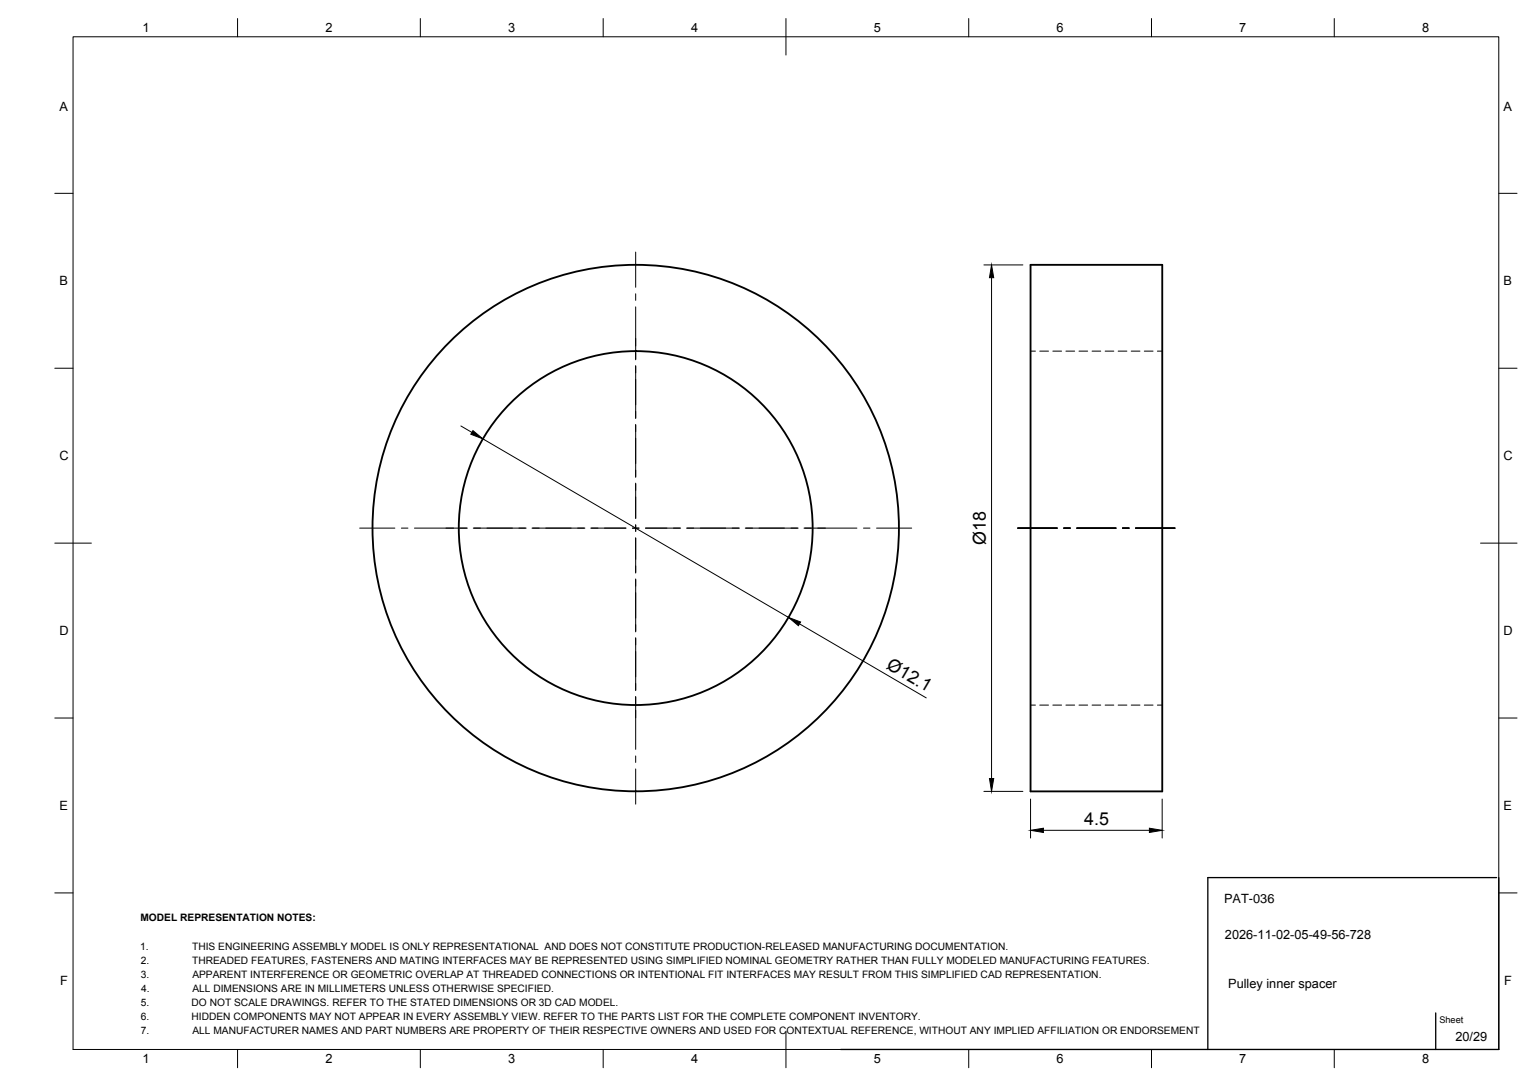
ISO-10303-21;
HEADER;
/* Generated by software containing ST-Developer
 * from STEP Tools, Inc. (www.steptools.com) 
 */

FILE_DESCRIPTION(
/* description */ ('Flange-mounted spindle'),
/* implementation_level */ '2;1');

FILE_NAME(
/* name */ 'Pulley inner spacer.step',
/* time_stamp */ '2026-10-27T10:49:51-07:00',
/* author */ (''),
/* organization */ (''),
/* preprocessor_version */ 'ST-DEVELOPER v20.2',
/* originating_system */ 'Autodesk Translation Framework v15.17.0.0',
/* authorisation */ '');

FILE_SCHEMA (('AUTOMOTIVE_DESIGN { 1 0 10303 214 3 1 1 }'));
ENDSEC;

DATA;
#10=MECHANICAL_DESIGN_GEOMETRIC_PRESENTATION_REPRESENTATION('',(#352),#11764);
#297=SHAPE_REPRESENTATION_RELATIONSHIP('SRR','None',#11895,#324);
#324=ADVANCED_BREP_SHAPE_REPRESENTATION('',(#378),#11750);
#352=STYLED_ITEM('',(#12113),#378);
#378=MANIFOLD_SOLID_BREP('Body1',#6146);
#457=FACE_BOUND('',#1228,.T.);
#458=FACE_BOUND('',#1230,.T.);
#594=PLANE('',#6714);
#595=PLANE('',#6715);
#814=FACE_OUTER_BOUND('',#1225,.T.);
#815=FACE_OUTER_BOUND('',#1226,.T.);
#816=FACE_OUTER_BOUND('',#1227,.T.);
#817=FACE_OUTER_BOUND('',#1229,.T.);
#1225=EDGE_LOOP('',(#4599,#4600,#4601,#4602));
#1226=EDGE_LOOP('',(#4603,#4604,#4605,#4606));
#1227=EDGE_LOOP('',(#4607));
#1228=EDGE_LOOP('',(#4608));
#1229=EDGE_LOOP('',(#4609));
#1230=EDGE_LOOP('',(#4610));
#1663=LINE('',#10200,#2085);
#1664=LINE('',#10206,#2086);
#2085=VECTOR('',#7894,0.605);
#2086=VECTOR('',#7901,0.9);
#2412=CIRCLE('',#6709,0.605);
#2413=CIRCLE('',#6710,0.605);
#2414=CIRCLE('',#6712,0.9);
#2415=CIRCLE('',#6713,0.9);
#2852=VERTEX_POINT('',#10197);
#2853=VERTEX_POINT('',#10199);
#2854=VERTEX_POINT('',#10203);
#2855=VERTEX_POINT('',#10205);
#3492=EDGE_CURVE('',#2852,#2852,#2412,.T.);
#3493=EDGE_CURVE('',#2852,#2853,#1663,.T.);
#3494=EDGE_CURVE('',#2853,#2853,#2413,.T.);
#3495=EDGE_CURVE('',#2854,#2854,#2414,.T.);
#3496=EDGE_CURVE('',#2854,#2855,#1664,.T.);
#3497=EDGE_CURVE('',#2855,#2855,#2415,.T.);
#4599=ORIENTED_EDGE('',*,*,#3492,.F.);
#4600=ORIENTED_EDGE('',*,*,#3493,.T.);
#4601=ORIENTED_EDGE('',*,*,#3494,.T.);
#4602=ORIENTED_EDGE('',*,*,#3493,.F.);
#4603=ORIENTED_EDGE('',*,*,#3495,.F.);
#4604=ORIENTED_EDGE('',*,*,#3496,.T.);
#4605=ORIENTED_EDGE('',*,*,#3497,.T.);
#4606=ORIENTED_EDGE('',*,*,#3496,.F.);
#4607=ORIENTED_EDGE('',*,*,#3495,.T.);
#4608=ORIENTED_EDGE('',*,*,#3492,.T.);
#4609=ORIENTED_EDGE('',*,*,#3497,.F.);
#4610=ORIENTED_EDGE('',*,*,#3494,.F.);
#5668=CYLINDRICAL_SURFACE('',#6708,0.605);
#5669=CYLINDRICAL_SURFACE('',#6711,0.9);
#5925=ADVANCED_FACE('',(#814),#5668,.F.);
#5926=ADVANCED_FACE('',(#815),#5669,.T.);
#5927=ADVANCED_FACE('',(#816,#457),#594,.T.);
#5928=ADVANCED_FACE('',(#817,#458),#595,.F.);
#6146=CLOSED_SHELL('',(#5925,#5926,#5927,#5928));
#6707=AXIS2_PLACEMENT_3D('',#10195,#7888,#7889);
#6708=AXIS2_PLACEMENT_3D('',#10196,#7890,#7891);
#6709=AXIS2_PLACEMENT_3D('',#10198,#7892,#7893);
#6710=AXIS2_PLACEMENT_3D('',#10201,#7895,#7896);
#6711=AXIS2_PLACEMENT_3D('',#10202,#7897,#7898);
#6712=AXIS2_PLACEMENT_3D('',#10204,#7899,#7900);
#6713=AXIS2_PLACEMENT_3D('',#10207,#7902,#7903);
#6714=AXIS2_PLACEMENT_3D('',#10208,#7904,#7905);
#6715=AXIS2_PLACEMENT_3D('',#10209,#7906,#7907);
#7888=DIRECTION('axis',(0.,0.,1.));
#7889=DIRECTION('refdir',(1.,0.,0.));
#7890=DIRECTION('center_axis',(0.,1.,0.));
#7891=DIRECTION('ref_axis',(1.,0.,0.));
#7892=DIRECTION('center_axis',(0.,-1.,0.));
#7893=DIRECTION('ref_axis',(1.,0.,0.));
#7894=DIRECTION('',(0.,-1.,0.));
#7895=DIRECTION('center_axis',(0.,-1.,0.));
#7896=DIRECTION('ref_axis',(1.,0.,0.));
#7897=DIRECTION('center_axis',(0.,1.,0.));
#7898=DIRECTION('ref_axis',(1.,0.,0.));
#7899=DIRECTION('center_axis',(0.,1.,0.));
#7900=DIRECTION('ref_axis',(1.,0.,0.));
#7901=DIRECTION('',(0.,-1.,0.));
#7902=DIRECTION('center_axis',(0.,1.,0.));
#7903=DIRECTION('ref_axis',(1.,0.,0.));
#7904=DIRECTION('center_axis',(0.,1.,0.));
#7905=DIRECTION('ref_axis',(1.,0.,0.));
#7906=DIRECTION('center_axis',(0.,1.,0.));
#7907=DIRECTION('ref_axis',(1.,0.,0.));
#10195=CARTESIAN_POINT('',(0.,0.,0.));
#10196=CARTESIAN_POINT('Origin',(0.,-4.95,8.));
#10197=CARTESIAN_POINT('',(-0.605,-4.5,8.));
#10198=CARTESIAN_POINT('Origin',(0.,-4.5,8.));
#10199=CARTESIAN_POINT('',(-0.605,-4.95,8.));
#10200=CARTESIAN_POINT('',(-0.605,-4.95,8.));
#10201=CARTESIAN_POINT('Origin',(0.,-4.95,8.));
#10202=CARTESIAN_POINT('Origin',(0.,-4.95,8.));
#10203=CARTESIAN_POINT('',(-0.9,-4.5,8.));
#10204=CARTESIAN_POINT('Origin',(0.,-4.5,8.));
#10205=CARTESIAN_POINT('',(-0.9,-4.95,8.));
#10206=CARTESIAN_POINT('',(-0.9,-4.95,8.));
#10207=CARTESIAN_POINT('Origin',(0.,-4.95,8.));
#10208=CARTESIAN_POINT('Origin',(0.,-4.5,8.));
#10209=CARTESIAN_POINT('Origin',(0.,-4.95,8.));
#11718=UNCERTAINTY_MEASURE_WITH_UNIT(LENGTH_MEASURE(0.001),#11765,
'DISTANCE_ACCURACY_VALUE',
'Maximum model space distance between geometric entities at asserted c
onnectivities');
#11732=UNCERTAINTY_MEASURE_WITH_UNIT(LENGTH_MEASURE(0.001),#11765,
'DISTANCE_ACCURACY_VALUE',
'Maximum model space distance between geometric entities at asserted c
onnectivities');
#11750=(
GEOMETRIC_REPRESENTATION_CONTEXT(3)
GLOBAL_UNCERTAINTY_ASSIGNED_CONTEXT((#11718))
GLOBAL_UNIT_ASSIGNED_CONTEXT((#11765,#11767,#11768))
REPRESENTATION_CONTEXT('','3D')
);
#11764=(
GEOMETRIC_REPRESENTATION_CONTEXT(3)
GLOBAL_UNCERTAINTY_ASSIGNED_CONTEXT((#11732))
GLOBAL_UNIT_ASSIGNED_CONTEXT((#11765,#11767,#11768))
REPRESENTATION_CONTEXT('','3D')
);
#11765=(
LENGTH_UNIT()
NAMED_UNIT(*)
SI_UNIT(.CENTI.,.METRE.)
);
#11767=(
NAMED_UNIT(*)
PLANE_ANGLE_UNIT()
SI_UNIT($,.RADIAN.)
);
#11768=(
NAMED_UNIT(*)
SI_UNIT($,.STERADIAN.)
SOLID_ANGLE_UNIT()
);
#11786=SHAPE_DEFINITION_REPRESENTATION(#11819,#11895);
#11819=PRODUCT_DEFINITION_SHAPE('',$,#11927);
#11895=SHAPE_REPRESENTATION('',(#6707),#11750);
#11909=PRODUCT_DEFINITION_CONTEXT('part definition',#12004,'design');
#11927=PRODUCT_DEFINITION('Pulley inner spacer','Pulley inner spacer',#11958,
#11909);
#11958=PRODUCT_DEFINITION_FORMATION('',$,#12023);
#12004=APPLICATION_CONTEXT(
'Core Data for Automotive Mechanical Design Process');
#12005=PRODUCT_CONTEXT('part definition',#12004,'mechanical');
#12023=PRODUCT('Pulley inner spacer','Pulley inner spacer',
'Pulley inner spacer',(#12005));
#12107=COLOUR_RGB('Off White',0.89,0.88,0.83);
#12108=FILL_AREA_STYLE_COLOUR('',#12107);
#12109=FILL_AREA_STYLE('',(#12108));
#12110=SURFACE_STYLE_FILL_AREA(#12109);
#12111=SURFACE_SIDE_STYLE('',(#12110));
#12112=SURFACE_STYLE_USAGE(.BOTH.,#12111);
#12113=PRESENTATION_STYLE_ASSIGNMENT((#12112));
ENDSEC;
END-ISO-10303-21;
